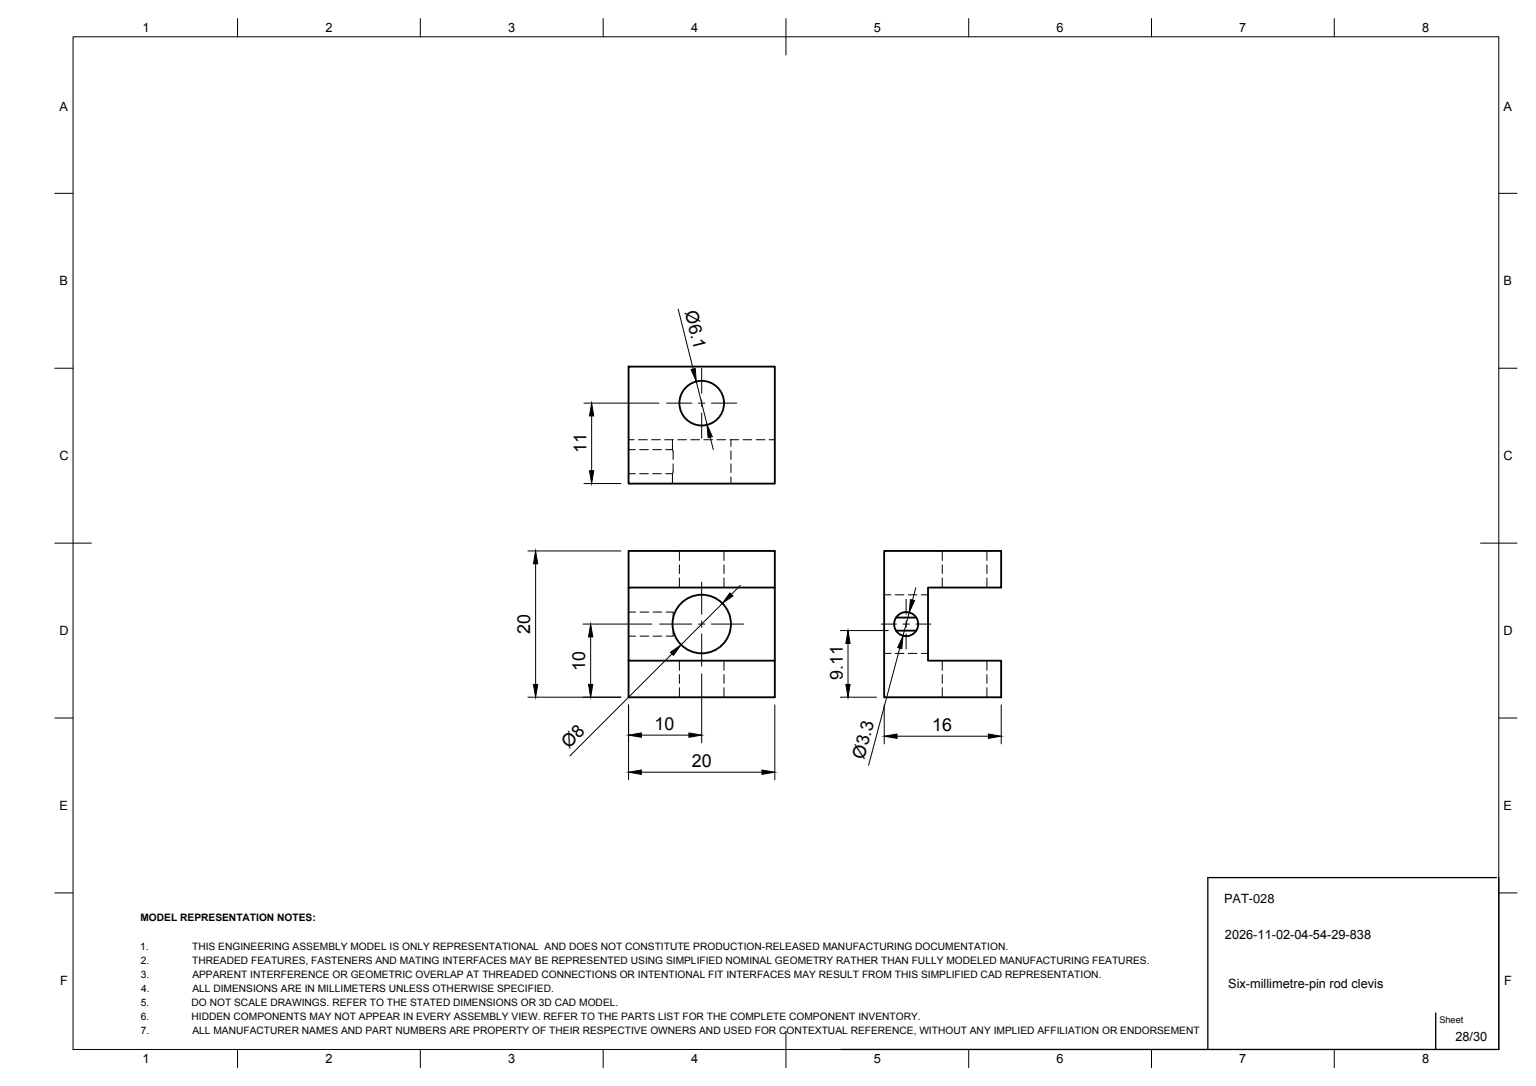
ISO-10303-21;
HEADER;
/* Generated by software containing ST-Developer
 * from STEP Tools, Inc. (www.steptools.com) 
 */

FILE_DESCRIPTION(
/* description */ ('Cylinder foot and clevis mount kit'),
/* implementation_level */ '2;1');

FILE_NAME(
/* name */ 'Six-millimetre-pin rod clevis.step',
/* time_stamp */ '2026-10-27T20:10:43-07:00',
/* author */ (''),
/* organization */ (''),
/* preprocessor_version */ 'ST-DEVELOPER v20.2',
/* originating_system */ 'Autodesk Translation Framework v15.17.0.0',
/* authorisation */ '');

FILE_SCHEMA (('AUTOMOTIVE_DESIGN { 1 0 10303 214 3 1 1 }'));
ENDSEC;

DATA;
#10=MECHANICAL_DESIGN_GEOMETRIC_PRESENTATION_REPRESENTATION('',(#361),#9102);
#11=B_SPLINE_CURVE_WITH_KNOTS('',3,(#8691,#8692,#8693,#8694,#8695,#8696,
#8697,#8698,#8699,#8700),.UNSPECIFIED.,.F.,.F.,(4,2,2,2,4),(0.665271585430998,
0.692803751398643,0.75574615888762,0.818688566376597,0.846220732344242),
 .UNSPECIFIED.);
#12=B_SPLINE_CURVE_WITH_KNOTS('',3,(#8708,#8709,#8710,#8711,#8712,#8713,
#8714,#8715,#8716,#8717),.UNSPECIFIED.,.F.,.F.,(4,2,2,2,4),(0.161440812839251,
0.188972978806896,0.251915386295873,0.31485779378485,0.342389959752495),
 .UNSPECIFIED.);
#305=SHAPE_REPRESENTATION_RELATIONSHIP('SRR','None',#9254,#333);
#333=ADVANCED_BREP_SHAPE_REPRESENTATION('',(#387),#9097);
#361=STYLED_ITEM('',(#9460),#387);
#387=MANIFOLD_SOLID_BREP('Body1',#4949);
#481=FACE_BOUND('',#1357,.T.);
#482=FACE_BOUND('',#1359,.T.);
#483=FACE_BOUND('',#1361,.T.);
#484=FACE_BOUND('',#1363,.T.);
#485=FACE_BOUND('',#1368,.T.);
#486=FACE_BOUND('',#1370,.T.);
#487=FACE_BOUND('',#1372,.T.);
#488=FACE_BOUND('',#1374,.T.);
#666=PLANE('',#5806);
#667=PLANE('',#5812);
#668=PLANE('',#5816);
#669=PLANE('',#5817);
#670=PLANE('',#5818);
#671=PLANE('',#5819);
#672=PLANE('',#5820);
#673=PLANE('',#5821);
#674=PLANE('',#5822);
#675=PLANE('',#5823);
#676=PLANE('',#5824);
#677=PLANE('',#5825);
#956=FACE_OUTER_BOUND('',#1351,.T.);
#957=FACE_OUTER_BOUND('',#1352,.T.);
#958=FACE_OUTER_BOUND('',#1353,.T.);
#959=FACE_OUTER_BOUND('',#1354,.T.);
#960=FACE_OUTER_BOUND('',#1355,.T.);
#961=FACE_OUTER_BOUND('',#1356,.T.);
#962=FACE_OUTER_BOUND('',#1358,.T.);
#963=FACE_OUTER_BOUND('',#1360,.T.);
#964=FACE_OUTER_BOUND('',#1362,.T.);
#965=FACE_OUTER_BOUND('',#1364,.T.);
#966=FACE_OUTER_BOUND('',#1365,.T.);
#967=FACE_OUTER_BOUND('',#1366,.T.);
#968=FACE_OUTER_BOUND('',#1367,.T.);
#969=FACE_OUTER_BOUND('',#1369,.T.);
#970=FACE_OUTER_BOUND('',#1371,.T.);
#971=FACE_OUTER_BOUND('',#1373,.T.);
#1351=EDGE_LOOP('',(#4319,#4320,#4321,#4322));
#1352=EDGE_LOOP('',(#4323,#4324,#4325,#4326));
#1353=EDGE_LOOP('',(#4327,#4328));
#1354=EDGE_LOOP('',(#4329,#4330,#4331,#4332,#4333,#4334,#4335,#4336));
#1355=EDGE_LOOP('',(#4337,#4338,#4339));
#1356=EDGE_LOOP('',(#4340,#4341,#4342,#4343));
#1357=EDGE_LOOP('',(#4344,#4345,#4346,#4347));
#1358=EDGE_LOOP('',(#4348,#4349,#4350,#4351));
#1359=EDGE_LOOP('',(#4352));
#1360=EDGE_LOOP('',(#4353,#4354,#4355,#4356));
#1361=EDGE_LOOP('',(#4357));
#1362=EDGE_LOOP('',(#4358,#4359,#4360,#4361));
#1363=EDGE_LOOP('',(#4362));
#1364=EDGE_LOOP('',(#4363,#4364,#4365,#4366,#4367,#4368,#4369,#4370));
#1365=EDGE_LOOP('',(#4371,#4372,#4373,#4374));
#1366=EDGE_LOOP('',(#4375,#4376,#4377,#4378));
#1367=EDGE_LOOP('',(#4379,#4380,#4381,#4382));
#1368=EDGE_LOOP('',(#4383));
#1369=EDGE_LOOP('',(#4384,#4385,#4386,#4387));
#1370=EDGE_LOOP('',(#4388));
#1371=EDGE_LOOP('',(#4389,#4390,#4391,#4392));
#1372=EDGE_LOOP('',(#4393));
#1373=EDGE_LOOP('',(#4394,#4395,#4396,#4397,#4398,#4399,#4400,#4401));
#1374=EDGE_LOOP('',(#4402));
#1695=LINE('',#8676,#2044);
#1696=LINE('',#8682,#2045);
#1697=LINE('',#8687,#2046);
#1698=LINE('',#8704,#2047);
#1699=LINE('',#8719,#2048);
#1700=LINE('',#8724,#2049);
#1701=LINE('',#8729,#2050);
#1702=LINE('',#8731,#2051);
#1703=LINE('',#8733,#2052);
#1704=LINE('',#8734,#2053);
#1705=LINE('',#8737,#2054);
#1706=LINE('',#8739,#2055);
#1707=LINE('',#8740,#2056);
#1708=LINE('',#8743,#2057);
#1709=LINE('',#8745,#2058);
#1710=LINE('',#8746,#2059);
#1711=LINE('',#8749,#2060);
#1712=LINE('',#8751,#2061);
#1713=LINE('',#8753,#2062);
#1714=LINE('',#8755,#2063);
#1715=LINE('',#8756,#2064);
#1716=LINE('',#8759,#2065);
#1717=LINE('',#8760,#2066);
#1718=LINE('',#8763,#2067);
#1719=LINE('',#8764,#2068);
#1720=LINE('',#8767,#2069);
#1721=LINE('',#8769,#2070);
#1722=LINE('',#8770,#2071);
#1723=LINE('',#8772,#2072);
#1724=LINE('',#8774,#2073);
#2044=VECTOR('',#7254,0.305);
#2045=VECTOR('',#7261,0.305);
#2046=VECTOR('',#7266,1.);
#2047=VECTOR('',#7273,0.165);
#2048=VECTOR('',#7280,1.);
#2049=VECTOR('',#7285,0.4);
#2050=VECTOR('',#7290,1.);
#2051=VECTOR('',#7291,1.);
#2052=VECTOR('',#7292,1.);
#2053=VECTOR('',#7293,1.);
#2054=VECTOR('',#7296,1.);
#2055=VECTOR('',#7297,1.);
#2056=VECTOR('',#7298,1.);
#2057=VECTOR('',#7301,1.);
#2058=VECTOR('',#7302,1.);
#2059=VECTOR('',#7303,1.);
#2060=VECTOR('',#7306,1.);
#2061=VECTOR('',#7307,1.);
#2062=VECTOR('',#7308,1.);
#2063=VECTOR('',#7309,1.);
#2064=VECTOR('',#7310,1.);
#2065=VECTOR('',#7313,1.);
#2066=VECTOR('',#7314,1.);
#2067=VECTOR('',#7317,1.);
#2068=VECTOR('',#7318,1.);
#2069=VECTOR('',#7321,1.);
#2070=VECTOR('',#7322,1.);
#2071=VECTOR('',#7323,1.);
#2072=VECTOR('',#7326,1.);
#2073=VECTOR('',#7329,1.);
#2299=CIRCLE('',#5801,0.305);
#2300=CIRCLE('',#5802,0.305);
#2301=CIRCLE('',#5804,0.305);
#2302=CIRCLE('',#5805,0.305);
#2303=CIRCLE('',#5807,0.165);
#2304=CIRCLE('',#5809,0.165);
#2305=CIRCLE('',#5810,0.165);
#2306=CIRCLE('',#5811,0.165);
#2307=CIRCLE('',#5814,0.4);
#2308=CIRCLE('',#5815,0.4);
#2646=VERTEX_POINT('',#8673);
#2647=VERTEX_POINT('',#8675);
#2648=VERTEX_POINT('',#8679);
#2649=VERTEX_POINT('',#8681);
#2650=VERTEX_POINT('',#8685);
#2651=VERTEX_POINT('',#8686);
#2652=VERTEX_POINT('',#8690);
#2653=VERTEX_POINT('',#8701);
#2654=VERTEX_POINT('',#8703);
#2655=VERTEX_POINT('',#8706);
#2656=VERTEX_POINT('',#8721);
#2657=VERTEX_POINT('',#8723);
#2658=VERTEX_POINT('',#8727);
#2659=VERTEX_POINT('',#8728);
#2660=VERTEX_POINT('',#8730);
#2661=VERTEX_POINT('',#8732);
#2662=VERTEX_POINT('',#8736);
#2663=VERTEX_POINT('',#8738);
#2664=VERTEX_POINT('',#8742);
#2665=VERTEX_POINT('',#8744);
#2666=VERTEX_POINT('',#8748);
#2667=VERTEX_POINT('',#8750);
#2668=VERTEX_POINT('',#8752);
#2669=VERTEX_POINT('',#8754);
#2670=VERTEX_POINT('',#8758);
#2671=VERTEX_POINT('',#8762);
#2672=VERTEX_POINT('',#8766);
#2673=VERTEX_POINT('',#8768);
#3214=EDGE_CURVE('',#2646,#2646,#2299,.T.);
#3215=EDGE_CURVE('',#2646,#2647,#1695,.T.);
#3216=EDGE_CURVE('',#2647,#2647,#2300,.T.);
#3217=EDGE_CURVE('',#2648,#2648,#2301,.T.);
#3218=EDGE_CURVE('',#2648,#2649,#1696,.T.);
#3219=EDGE_CURVE('',#2649,#2649,#2302,.T.);
#3220=EDGE_CURVE('',#2650,#2651,#1697,.T.);
#3221=EDGE_CURVE('',#2650,#2651,#2303,.T.);
#3222=EDGE_CURVE('',#2652,#2650,#11,.T.);
#3223=EDGE_CURVE('',#2653,#2652,#2304,.T.);
#3224=EDGE_CURVE('',#2653,#2654,#1698,.T.);
#3225=EDGE_CURVE('',#2654,#2654,#2305,.T.);
#3226=EDGE_CURVE('',#2655,#2653,#2306,.T.);
#3227=EDGE_CURVE('',#2651,#2655,#12,.T.);
#3228=EDGE_CURVE('',#2655,#2652,#1699,.T.);
#3229=EDGE_CURVE('',#2656,#2656,#2307,.T.);
#3230=EDGE_CURVE('',#2656,#2657,#1700,.T.);
#3231=EDGE_CURVE('',#2657,#2657,#2308,.T.);
#3232=EDGE_CURVE('',#2658,#2659,#1701,.T.);
#3233=EDGE_CURVE('',#2660,#2658,#1702,.T.);
#3234=EDGE_CURVE('',#2661,#2660,#1703,.T.);
#3235=EDGE_CURVE('',#2659,#2661,#1704,.T.);
#3236=EDGE_CURVE('',#2662,#2658,#1705,.T.);
#3237=EDGE_CURVE('',#2663,#2662,#1706,.T.);
#3238=EDGE_CURVE('',#2660,#2663,#1707,.T.);
#3239=EDGE_CURVE('',#2664,#2662,#1708,.T.);
#3240=EDGE_CURVE('',#2665,#2664,#1709,.T.);
#3241=EDGE_CURVE('',#2663,#2665,#1710,.T.);
#3242=EDGE_CURVE('',#2666,#2665,#1711,.T.);
#3243=EDGE_CURVE('',#2667,#2666,#1712,.T.);
#3244=EDGE_CURVE('',#2668,#2667,#1713,.T.);
#3245=EDGE_CURVE('',#2669,#2668,#1714,.T.);
#3246=EDGE_CURVE('',#2661,#2669,#1715,.T.);
#3247=EDGE_CURVE('',#2670,#2664,#1716,.T.);
#3248=EDGE_CURVE('',#2666,#2670,#1717,.T.);
#3249=EDGE_CURVE('',#2669,#2671,#1718,.T.);
#3250=EDGE_CURVE('',#2659,#2671,#1719,.T.);
#3251=EDGE_CURVE('',#2667,#2672,#1720,.T.);
#3252=EDGE_CURVE('',#2673,#2672,#1721,.T.);
#3253=EDGE_CURVE('',#2668,#2673,#1722,.T.);
#3254=EDGE_CURVE('',#2671,#2673,#1723,.T.);
#3255=EDGE_CURVE('',#2672,#2670,#1724,.T.);
#4319=ORIENTED_EDGE('',*,*,#3214,.F.);
#4320=ORIENTED_EDGE('',*,*,#3215,.T.);
#4321=ORIENTED_EDGE('',*,*,#3216,.F.);
#4322=ORIENTED_EDGE('',*,*,#3215,.F.);
#4323=ORIENTED_EDGE('',*,*,#3217,.F.);
#4324=ORIENTED_EDGE('',*,*,#3218,.T.);
#4325=ORIENTED_EDGE('',*,*,#3219,.F.);
#4326=ORIENTED_EDGE('',*,*,#3218,.F.);
#4327=ORIENTED_EDGE('',*,*,#3220,.F.);
#4328=ORIENTED_EDGE('',*,*,#3221,.T.);
#4329=ORIENTED_EDGE('',*,*,#3222,.F.);
#4330=ORIENTED_EDGE('',*,*,#3223,.F.);
#4331=ORIENTED_EDGE('',*,*,#3224,.T.);
#4332=ORIENTED_EDGE('',*,*,#3225,.F.);
#4333=ORIENTED_EDGE('',*,*,#3224,.F.);
#4334=ORIENTED_EDGE('',*,*,#3226,.F.);
#4335=ORIENTED_EDGE('',*,*,#3227,.F.);
#4336=ORIENTED_EDGE('',*,*,#3221,.F.);
#4337=ORIENTED_EDGE('',*,*,#3228,.F.);
#4338=ORIENTED_EDGE('',*,*,#3226,.T.);
#4339=ORIENTED_EDGE('',*,*,#3223,.T.);
#4340=ORIENTED_EDGE('',*,*,#3229,.F.);
#4341=ORIENTED_EDGE('',*,*,#3230,.T.);
#4342=ORIENTED_EDGE('',*,*,#3231,.F.);
#4343=ORIENTED_EDGE('',*,*,#3230,.F.);
#4344=ORIENTED_EDGE('',*,*,#3227,.T.);
#4345=ORIENTED_EDGE('',*,*,#3228,.T.);
#4346=ORIENTED_EDGE('',*,*,#3222,.T.);
#4347=ORIENTED_EDGE('',*,*,#3220,.T.);
#4348=ORIENTED_EDGE('',*,*,#3232,.F.);
#4349=ORIENTED_EDGE('',*,*,#3233,.F.);
#4350=ORIENTED_EDGE('',*,*,#3234,.F.);
#4351=ORIENTED_EDGE('',*,*,#3235,.F.);
#4352=ORIENTED_EDGE('',*,*,#3217,.T.);
#4353=ORIENTED_EDGE('',*,*,#3236,.F.);
#4354=ORIENTED_EDGE('',*,*,#3237,.F.);
#4355=ORIENTED_EDGE('',*,*,#3238,.F.);
#4356=ORIENTED_EDGE('',*,*,#3233,.T.);
#4357=ORIENTED_EDGE('',*,*,#3229,.T.);
#4358=ORIENTED_EDGE('',*,*,#3239,.F.);
#4359=ORIENTED_EDGE('',*,*,#3240,.F.);
#4360=ORIENTED_EDGE('',*,*,#3241,.F.);
#4361=ORIENTED_EDGE('',*,*,#3237,.T.);
#4362=ORIENTED_EDGE('',*,*,#3216,.T.);
#4363=ORIENTED_EDGE('',*,*,#3234,.T.);
#4364=ORIENTED_EDGE('',*,*,#3238,.T.);
#4365=ORIENTED_EDGE('',*,*,#3241,.T.);
#4366=ORIENTED_EDGE('',*,*,#3242,.F.);
#4367=ORIENTED_EDGE('',*,*,#3243,.F.);
#4368=ORIENTED_EDGE('',*,*,#3244,.F.);
#4369=ORIENTED_EDGE('',*,*,#3245,.F.);
#4370=ORIENTED_EDGE('',*,*,#3246,.F.);
#4371=ORIENTED_EDGE('',*,*,#3240,.T.);
#4372=ORIENTED_EDGE('',*,*,#3247,.F.);
#4373=ORIENTED_EDGE('',*,*,#3248,.F.);
#4374=ORIENTED_EDGE('',*,*,#3242,.T.);
#4375=ORIENTED_EDGE('',*,*,#3235,.T.);
#4376=ORIENTED_EDGE('',*,*,#3246,.T.);
#4377=ORIENTED_EDGE('',*,*,#3249,.T.);
#4378=ORIENTED_EDGE('',*,*,#3250,.F.);
#4379=ORIENTED_EDGE('',*,*,#3244,.T.);
#4380=ORIENTED_EDGE('',*,*,#3251,.T.);
#4381=ORIENTED_EDGE('',*,*,#3252,.F.);
#4382=ORIENTED_EDGE('',*,*,#3253,.F.);
#4383=ORIENTED_EDGE('',*,*,#3231,.T.);
#4384=ORIENTED_EDGE('',*,*,#3245,.T.);
#4385=ORIENTED_EDGE('',*,*,#3253,.T.);
#4386=ORIENTED_EDGE('',*,*,#3254,.F.);
#4387=ORIENTED_EDGE('',*,*,#3249,.F.);
#4388=ORIENTED_EDGE('',*,*,#3219,.T.);
#4389=ORIENTED_EDGE('',*,*,#3243,.T.);
#4390=ORIENTED_EDGE('',*,*,#3248,.T.);
#4391=ORIENTED_EDGE('',*,*,#3255,.F.);
#4392=ORIENTED_EDGE('',*,*,#3251,.F.);
#4393=ORIENTED_EDGE('',*,*,#3214,.T.);
#4394=ORIENTED_EDGE('',*,*,#3232,.T.);
#4395=ORIENTED_EDGE('',*,*,#3250,.T.);
#4396=ORIENTED_EDGE('',*,*,#3254,.T.);
#4397=ORIENTED_EDGE('',*,*,#3252,.T.);
#4398=ORIENTED_EDGE('',*,*,#3255,.T.);
#4399=ORIENTED_EDGE('',*,*,#3247,.T.);
#4400=ORIENTED_EDGE('',*,*,#3239,.T.);
#4401=ORIENTED_EDGE('',*,*,#3236,.T.);
#4402=ORIENTED_EDGE('',*,*,#3225,.T.);
#4607=CYLINDRICAL_SURFACE('',#5800,0.305);
#4608=CYLINDRICAL_SURFACE('',#5803,0.305);
#4609=CYLINDRICAL_SURFACE('',#5808,0.165);
#4610=CYLINDRICAL_SURFACE('',#5813,0.4);
#4879=ADVANCED_FACE('',(#956),#4607,.F.);
#4880=ADVANCED_FACE('',(#957),#4608,.F.);
#4881=ADVANCED_FACE('',(#958),#666,.T.);
#4882=ADVANCED_FACE('',(#959),#4609,.F.);
#4883=ADVANCED_FACE('',(#960),#667,.T.);
#4884=ADVANCED_FACE('',(#961,#481),#4610,.F.);
#4885=ADVANCED_FACE('',(#962,#482),#668,.F.);
#4886=ADVANCED_FACE('',(#963,#483),#669,.F.);
#4887=ADVANCED_FACE('',(#964,#484),#670,.F.);
#4888=ADVANCED_FACE('',(#965),#671,.F.);
#4889=ADVANCED_FACE('',(#966),#672,.T.);
#4890=ADVANCED_FACE('',(#967),#673,.T.);
#4891=ADVANCED_FACE('',(#968,#485),#674,.T.);
#4892=ADVANCED_FACE('',(#969,#486),#675,.T.);
#4893=ADVANCED_FACE('',(#970,#487),#676,.T.);
#4894=ADVANCED_FACE('',(#971,#488),#677,.T.);
#4949=CLOSED_SHELL('',(#4879,#4880,#4881,#4882,#4883,#4884,#4885,#4886,
#4887,#4888,#4889,#4890,#4891,#4892,#4893,#4894));
#5799=AXIS2_PLACEMENT_3D('',#8671,#7248,#7249);
#5800=AXIS2_PLACEMENT_3D('',#8672,#7250,#7251);
#5801=AXIS2_PLACEMENT_3D('',#8674,#7252,#7253);
#5802=AXIS2_PLACEMENT_3D('',#8677,#7255,#7256);
#5803=AXIS2_PLACEMENT_3D('',#8678,#7257,#7258);
#5804=AXIS2_PLACEMENT_3D('',#8680,#7259,#7260);
#5805=AXIS2_PLACEMENT_3D('',#8683,#7262,#7263);
#5806=AXIS2_PLACEMENT_3D('',#8684,#7264,#7265);
#5807=AXIS2_PLACEMENT_3D('',#8688,#7267,#7268);
#5808=AXIS2_PLACEMENT_3D('',#8689,#7269,#7270);
#5809=AXIS2_PLACEMENT_3D('',#8702,#7271,#7272);
#5810=AXIS2_PLACEMENT_3D('',#8705,#7274,#7275);
#5811=AXIS2_PLACEMENT_3D('',#8707,#7276,#7277);
#5812=AXIS2_PLACEMENT_3D('',#8718,#7278,#7279);
#5813=AXIS2_PLACEMENT_3D('',#8720,#7281,#7282);
#5814=AXIS2_PLACEMENT_3D('',#8722,#7283,#7284);
#5815=AXIS2_PLACEMENT_3D('',#8725,#7286,#7287);
#5816=AXIS2_PLACEMENT_3D('',#8726,#7288,#7289);
#5817=AXIS2_PLACEMENT_3D('',#8735,#7294,#7295);
#5818=AXIS2_PLACEMENT_3D('',#8741,#7299,#7300);
#5819=AXIS2_PLACEMENT_3D('',#8747,#7304,#7305);
#5820=AXIS2_PLACEMENT_3D('',#8757,#7311,#7312);
#5821=AXIS2_PLACEMENT_3D('',#8761,#7315,#7316);
#5822=AXIS2_PLACEMENT_3D('',#8765,#7319,#7320);
#5823=AXIS2_PLACEMENT_3D('',#8771,#7324,#7325);
#5824=AXIS2_PLACEMENT_3D('',#8773,#7327,#7328);
#5825=AXIS2_PLACEMENT_3D('',#8775,#7330,#7331);
#7248=DIRECTION('axis',(0.,0.,1.));
#7249=DIRECTION('refdir',(1.,0.,0.));
#7250=DIRECTION('center_axis',(1.,0.,0.));
#7251=DIRECTION('ref_axis',(0.,0.,-1.));
#7252=DIRECTION('center_axis',(1.,0.,0.));
#7253=DIRECTION('ref_axis',(0.,0.,-1.));
#7254=DIRECTION('',(1.,0.,0.));
#7255=DIRECTION('center_axis',(-1.,0.,0.));
#7256=DIRECTION('ref_axis',(0.,0.,-1.));
#7257=DIRECTION('center_axis',(1.,0.,0.));
#7258=DIRECTION('ref_axis',(0.,0.,-1.));
#7259=DIRECTION('center_axis',(1.,0.,0.));
#7260=DIRECTION('ref_axis',(0.,0.,-1.));
#7261=DIRECTION('',(1.,0.,0.));
#7262=DIRECTION('center_axis',(-1.,0.,0.));
#7263=DIRECTION('ref_axis',(0.,0.,-1.));
#7264=DIRECTION('center_axis',(0.,0.,1.));
#7265=DIRECTION('ref_axis',(1.,0.,0.));
#7266=DIRECTION('',(0.,1.,0.));
#7267=DIRECTION('center_axis',(0.,0.,1.));
#7268=DIRECTION('ref_axis',(1.,0.,0.));
#7269=DIRECTION('center_axis',(0.,0.,1.));
#7270=DIRECTION('ref_axis',(1.,0.,0.));
#7271=DIRECTION('center_axis',(0.,0.,1.));
#7272=DIRECTION('ref_axis',(1.,0.,0.));
#7273=DIRECTION('',(0.,0.,1.));
#7274=DIRECTION('center_axis',(0.,0.,-1.));
#7275=DIRECTION('ref_axis',(1.,0.,0.));
#7276=DIRECTION('center_axis',(0.,0.,1.));
#7277=DIRECTION('ref_axis',(1.,0.,0.));
#7278=DIRECTION('center_axis',(0.,0.,1.));
#7279=DIRECTION('ref_axis',(1.,0.,0.));
#7280=DIRECTION('',(0.,-1.,0.));
#7281=DIRECTION('center_axis',(0.,1.,0.));
#7282=DIRECTION('ref_axis',(1.,0.,0.));
#7283=DIRECTION('center_axis',(0.,1.,0.));
#7284=DIRECTION('ref_axis',(1.,0.,0.));
#7285=DIRECTION('',(0.,1.,0.));
#7286=DIRECTION('center_axis',(0.,-1.,0.));
#7287=DIRECTION('ref_axis',(1.,0.,0.));
#7288=DIRECTION('center_axis',(1.,0.,0.));
#7289=DIRECTION('ref_axis',(0.,1.,0.));
#7290=DIRECTION('',(0.,-1.,0.));
#7291=DIRECTION('',(0.,0.,1.));
#7292=DIRECTION('',(0.,1.,0.));
#7293=DIRECTION('',(0.,0.,-1.));
#7294=DIRECTION('center_axis',(0.,1.,0.));
#7295=DIRECTION('ref_axis',(-1.,0.,0.));
#7296=DIRECTION('',(1.,0.,0.));
#7297=DIRECTION('',(0.,0.,1.));
#7298=DIRECTION('',(-1.,0.,0.));
#7299=DIRECTION('center_axis',(-1.,0.,0.));
#7300=DIRECTION('ref_axis',(0.,-1.,0.));
#7301=DIRECTION('',(0.,1.,0.));
#7302=DIRECTION('',(0.,0.,1.));
#7303=DIRECTION('',(0.,-1.,0.));
#7304=DIRECTION('center_axis',(0.,0.,1.));
#7305=DIRECTION('ref_axis',(1.,0.,0.));
#7306=DIRECTION('',(1.,0.,0.));
#7307=DIRECTION('',(0.,-1.,0.));
#7308=DIRECTION('',(-1.,0.,0.));
#7309=DIRECTION('',(0.,1.,0.));
#7310=DIRECTION('',(1.,0.,0.));
#7311=DIRECTION('center_axis',(0.,-1.,0.));
#7312=DIRECTION('ref_axis',(1.,0.,0.));
#7313=DIRECTION('',(1.,0.,0.));
#7314=DIRECTION('',(0.,0.,1.));
#7315=DIRECTION('center_axis',(0.,-1.,0.));
#7316=DIRECTION('ref_axis',(1.,0.,0.));
#7317=DIRECTION('',(0.,0.,1.));
#7318=DIRECTION('',(1.,0.,0.));
#7319=DIRECTION('center_axis',(0.,1.,0.));
#7320=DIRECTION('ref_axis',(-1.,0.,0.));
#7321=DIRECTION('',(0.,0.,1.));
#7322=DIRECTION('',(-1.,0.,0.));
#7323=DIRECTION('',(0.,0.,1.));
#7324=DIRECTION('center_axis',(1.,0.,0.));
#7325=DIRECTION('ref_axis',(0.,1.,0.));
#7326=DIRECTION('',(0.,1.,0.));
#7327=DIRECTION('center_axis',(-1.,0.,0.));
#7328=DIRECTION('ref_axis',(0.,-1.,0.));
#7329=DIRECTION('',(0.,-1.,0.));
#7330=DIRECTION('center_axis',(0.,0.,1.));
#7331=DIRECTION('ref_axis',(1.,0.,0.));
#8671=CARTESIAN_POINT('',(0.,0.,0.));
#8672=CARTESIAN_POINT('Origin',(-1.1,-6.1,4.5));
#8673=CARTESIAN_POINT('',(-1.,-6.1,4.805));
#8674=CARTESIAN_POINT('Origin',(-1.,-6.1,4.5));
#8675=CARTESIAN_POINT('',(-0.5,-6.1,4.805));
#8676=CARTESIAN_POINT('',(-1.1,-6.1,4.805));
#8677=CARTESIAN_POINT('Origin',(-0.5,-6.1,4.5));
#8678=CARTESIAN_POINT('Origin',(-1.1,-6.1,4.5));
#8679=CARTESIAN_POINT('',(0.5,-6.1,4.805));
#8680=CARTESIAN_POINT('Origin',(0.5,-6.1,4.5));
#8681=CARTESIAN_POINT('',(1.,-6.1,4.805));
#8682=CARTESIAN_POINT('',(-1.1,-6.1,4.805));
#8683=CARTESIAN_POINT('Origin',(1.,-6.1,4.5));
#8684=CARTESIAN_POINT('Origin',(0.,-5.3,4.89));
#8685=CARTESIAN_POINT('',(0.0888819441731535,-5.43901438774458,4.89));
#8686=CARTESIAN_POINT('',(0.0888819441731535,-5.16098561225542,4.89));
#8687=CARTESIAN_POINT('',(0.0888819441731535,-5.6,4.89));
#8688=CARTESIAN_POINT('Origin',(0.,-5.3,4.89));
#8689=CARTESIAN_POINT('Origin',(0.,-5.3,4.89));
#8690=CARTESIAN_POINT('',(-0.0888819441731535,-5.43901438774458,4.89));
#8691=CARTESIAN_POINT('Ctrl Pts',(-0.0888819441731541,-5.43901438774458,
4.89));
#8692=CARTESIAN_POINT('Ctrl Pts',(-0.0808964434200148,-5.44412009546053,
4.89181991495419));
#8693=CARTESIAN_POINT('Ctrl Pts',(-0.0723643333023662,-5.44859639186021,
4.89350251788328));
#8694=CARTESIAN_POINT('Ctrl Pts',(-0.0431949313468613,-5.46075622416973,
4.89819171553211));
#8695=CARTESIAN_POINT('Ctrl Pts',(-0.0209808024963256,-5.465,4.9));
#8696=CARTESIAN_POINT('Ctrl Pts',(0.0209808024963256,-5.465,4.9));
#8697=CARTESIAN_POINT('Ctrl Pts',(0.0431949313468613,-5.46075622416973,
4.89819171553211));
#8698=CARTESIAN_POINT('Ctrl Pts',(0.0723643333023662,-5.44859639186021,
4.89350251788328));
#8699=CARTESIAN_POINT('Ctrl Pts',(0.0808964434200144,-5.44412009546053,
4.89181991495419));
#8700=CARTESIAN_POINT('Ctrl Pts',(0.0888819441731541,-5.43901438774458,
4.89));
#8701=CARTESIAN_POINT('',(-0.165,-5.3,4.89));
#8702=CARTESIAN_POINT('Origin',(0.,-5.3,4.89));
#8703=CARTESIAN_POINT('',(-0.165,-5.3,5.5));
#8704=CARTESIAN_POINT('',(-0.165,-5.3,4.89));
#8705=CARTESIAN_POINT('Origin',(0.,-5.3,5.5));
#8706=CARTESIAN_POINT('',(-0.0888819441731535,-5.16098561225542,4.89));
#8707=CARTESIAN_POINT('Origin',(0.,-5.3,4.89));
#8708=CARTESIAN_POINT('Ctrl Pts',(0.0888819441731536,-5.16098561225542,
4.89));
#8709=CARTESIAN_POINT('Ctrl Pts',(0.0808964434200141,-5.15587990453947,
4.89181991495419));
#8710=CARTESIAN_POINT('Ctrl Pts',(0.0723643333023662,-5.15140360813979,
4.89350251788328));
#8711=CARTESIAN_POINT('Ctrl Pts',(0.0431949313468613,-5.13924377583027,
4.89819171553211));
#8712=CARTESIAN_POINT('Ctrl Pts',(0.0209808024963256,-5.135,4.9));
#8713=CARTESIAN_POINT('Ctrl Pts',(-0.0209808024963256,-5.135,4.9));
#8714=CARTESIAN_POINT('Ctrl Pts',(-0.0431949313468613,-5.13924377583027,
4.89819171553211));
#8715=CARTESIAN_POINT('Ctrl Pts',(-0.0723643333023663,-5.15140360813979,
4.89350251788328));
#8716=CARTESIAN_POINT('Ctrl Pts',(-0.0808964434200144,-5.15587990453947,
4.89181991495419));
#8717=CARTESIAN_POINT('Ctrl Pts',(-0.0888819441731536,-5.16098561225542,
4.89));
#8718=CARTESIAN_POINT('Origin',(0.,-5.3,4.89));
#8719=CARTESIAN_POINT('',(-0.0888819441731535,-5.6,4.89));
#8720=CARTESIAN_POINT('Origin',(0.,-5.6,4.5));
#8721=CARTESIAN_POINT('',(-0.4,-5.6,4.5));
#8722=CARTESIAN_POINT('Origin',(0.,-5.6,4.5));
#8723=CARTESIAN_POINT('',(-0.4,-5.,4.5));
#8724=CARTESIAN_POINT('',(-0.4,-5.6,4.5));
#8725=CARTESIAN_POINT('Origin',(0.,-5.,4.5));
#8726=CARTESIAN_POINT('Origin',(0.5,-6.7,3.4));
#8727=CARTESIAN_POINT('',(0.5,-5.6,5.5));
#8728=CARTESIAN_POINT('',(0.5,-6.6,5.5));
#8729=CARTESIAN_POINT('',(0.5,-6.25,5.5));
#8730=CARTESIAN_POINT('',(0.5,-5.6,3.5));
#8731=CARTESIAN_POINT('',(0.5,-5.6,3.4));
#8732=CARTESIAN_POINT('',(0.5,-6.6,3.5));
#8733=CARTESIAN_POINT('',(0.5,-6.25,3.5));
#8734=CARTESIAN_POINT('',(0.5,-6.6,3.45));
#8735=CARTESIAN_POINT('Origin',(0.5,-5.6,3.4));
#8736=CARTESIAN_POINT('',(-0.5,-5.6,5.5));
#8737=CARTESIAN_POINT('',(0.25,-5.6,5.5));
#8738=CARTESIAN_POINT('',(-0.5,-5.6,3.5));
#8739=CARTESIAN_POINT('',(-0.5,-5.6,3.4));
#8740=CARTESIAN_POINT('',(0.25,-5.6,3.5));
#8741=CARTESIAN_POINT('Origin',(-0.5,-5.6,3.4));
#8742=CARTESIAN_POINT('',(-0.5,-6.6,5.5));
#8743=CARTESIAN_POINT('',(-0.5,-5.7,5.5));
#8744=CARTESIAN_POINT('',(-0.5,-6.6,3.5));
#8745=CARTESIAN_POINT('',(-0.5,-6.6,3.45));
#8746=CARTESIAN_POINT('',(-0.5,-5.7,3.5));
#8747=CARTESIAN_POINT('Origin',(0.,-5.8,3.5));
#8748=CARTESIAN_POINT('',(-1.,-6.6,3.5));
#8749=CARTESIAN_POINT('',(-1.,-6.6,3.5));
#8750=CARTESIAN_POINT('',(-1.,-5.,3.5));
#8751=CARTESIAN_POINT('',(-1.,-5.,3.5));
#8752=CARTESIAN_POINT('',(1.,-5.,3.5));
#8753=CARTESIAN_POINT('',(1.,-5.,3.5));
#8754=CARTESIAN_POINT('',(1.,-6.6,3.5));
#8755=CARTESIAN_POINT('',(1.,-6.6,3.5));
#8756=CARTESIAN_POINT('',(-1.,-6.6,3.5));
#8757=CARTESIAN_POINT('Origin',(-1.,-6.6,3.5));
#8758=CARTESIAN_POINT('',(-1.,-6.6,5.5));
#8759=CARTESIAN_POINT('',(-1.,-6.6,5.5));
#8760=CARTESIAN_POINT('',(-1.,-6.6,3.5));
#8761=CARTESIAN_POINT('Origin',(-1.,-6.6,3.5));
#8762=CARTESIAN_POINT('',(1.,-6.6,5.5));
#8763=CARTESIAN_POINT('',(1.,-6.6,3.5));
#8764=CARTESIAN_POINT('',(-1.,-6.6,5.5));
#8765=CARTESIAN_POINT('Origin',(1.,-5.,3.5));
#8766=CARTESIAN_POINT('',(-1.,-5.,5.5));
#8767=CARTESIAN_POINT('',(-1.,-5.,3.5));
#8768=CARTESIAN_POINT('',(1.,-5.,5.5));
#8769=CARTESIAN_POINT('',(1.,-5.,5.5));
#8770=CARTESIAN_POINT('',(1.,-5.,3.5));
#8771=CARTESIAN_POINT('Origin',(1.,-6.6,3.5));
#8772=CARTESIAN_POINT('',(1.,-6.6,5.5));
#8773=CARTESIAN_POINT('Origin',(-1.,-5.,3.5));
#8774=CARTESIAN_POINT('',(-1.,-5.,5.5));
#8775=CARTESIAN_POINT('Origin',(0.,-5.8,5.5));
#9064=UNCERTAINTY_MEASURE_WITH_UNIT(LENGTH_MEASURE(0.001),#9103,
'DISTANCE_ACCURACY_VALUE',
'Maximum model space distance between geometric entities at asserted c
onnectivities');
#9069=UNCERTAINTY_MEASURE_WITH_UNIT(LENGTH_MEASURE(0.001),#9103,
'DISTANCE_ACCURACY_VALUE',
'Maximum model space distance between geometric entities at asserted c
onnectivities');
#9097=(
GEOMETRIC_REPRESENTATION_CONTEXT(3)
GLOBAL_UNCERTAINTY_ASSIGNED_CONTEXT((#9064))
GLOBAL_UNIT_ASSIGNED_CONTEXT((#9103,#9105,#9106))
REPRESENTATION_CONTEXT('','3D')
);
#9102=(
GEOMETRIC_REPRESENTATION_CONTEXT(3)
GLOBAL_UNCERTAINTY_ASSIGNED_CONTEXT((#9069))
GLOBAL_UNIT_ASSIGNED_CONTEXT((#9103,#9105,#9106))
REPRESENTATION_CONTEXT('','3D')
);
#9103=(
LENGTH_UNIT()
NAMED_UNIT(*)
SI_UNIT(.CENTI.,.METRE.)
);
#9105=(
NAMED_UNIT(*)
PLANE_ANGLE_UNIT()
SI_UNIT($,.RADIAN.)
);
#9106=(
NAMED_UNIT(*)
SI_UNIT($,.STERADIAN.)
SOLID_ANGLE_UNIT()
);
#9134=SHAPE_DEFINITION_REPRESENTATION(#9209,#9254);
#9209=PRODUCT_DEFINITION_SHAPE('',$,#9287);
#9254=SHAPE_REPRESENTATION('',(#5799),#9097);
#9259=PRODUCT_DEFINITION_CONTEXT('part definition',#9357,'design');
#9287=PRODUCT_DEFINITION('Six-millimetre-pin rod clevis',
'Six-millimetre-pin rod clevis',#9319,#9259);
#9319=PRODUCT_DEFINITION_FORMATION('',$,#9386);
#9357=APPLICATION_CONTEXT(
'Core Data for Automotive Mechanical Design Process');
#9358=PRODUCT_CONTEXT('part definition',#9357,'mechanical');
#9386=PRODUCT('Six-millimetre-pin rod clevis',
'Six-millimetre-pin rod clevis','Six-millimetre-pin rod clevis',(#9358));
#9454=COLOUR_RGB('Grey',0.48,0.52,0.57);
#9455=FILL_AREA_STYLE_COLOUR('',#9454);
#9456=FILL_AREA_STYLE('',(#9455));
#9457=SURFACE_STYLE_FILL_AREA(#9456);
#9458=SURFACE_SIDE_STYLE('',(#9457));
#9459=SURFACE_STYLE_USAGE(.BOTH.,#9458);
#9460=PRESENTATION_STYLE_ASSIGNMENT((#9459));
ENDSEC;
END-ISO-10303-21;
